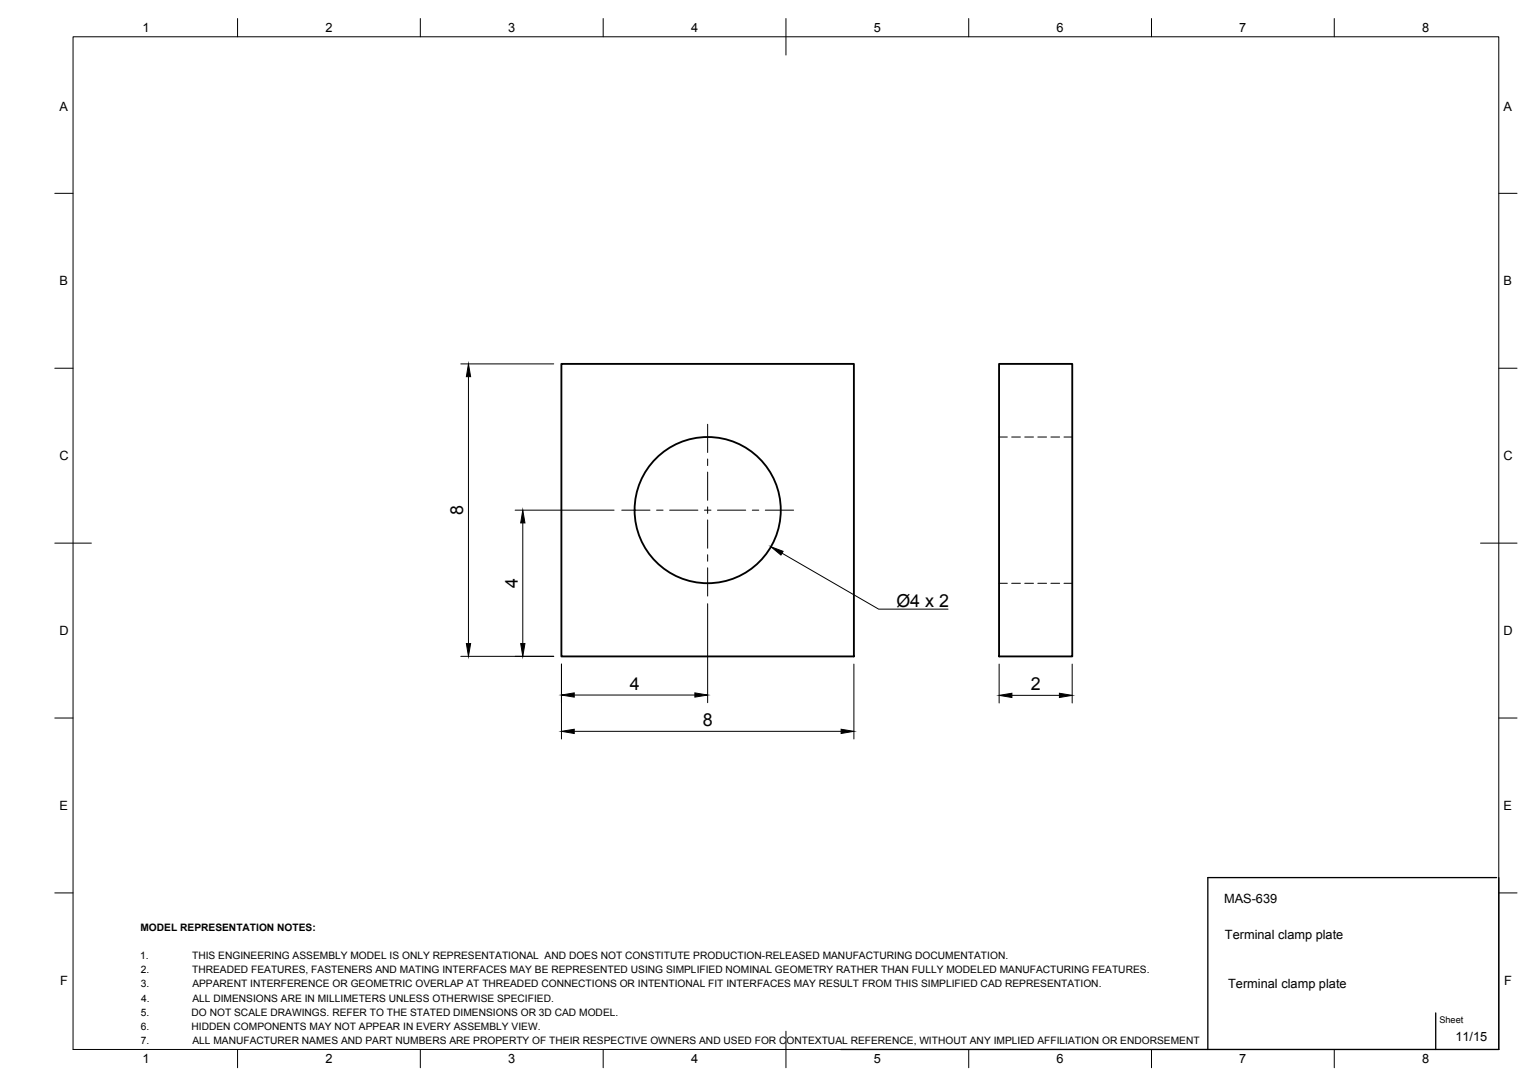
ISO-10303-21;
HEADER;
/* Generated by software containing ST-Developer
 * from STEP Tools, Inc. (www.steptools.com) 
 */

FILE_DESCRIPTION(
/* description */ ('Independent maintained push-to-latch/pull-to-reset mushroom-operator 
CAD. Two opposed spring-loaded ball detents in turned circular seats b
ias both travel stops; direct normally-closed bridge opens6mm when pre
ssed. Rounded palm/pull rim, captured head screw, removable detent clo
sures, native Coil spring families, insulated shared terminals and ord
inary machining features. Manual geometric states and ideal same-mater
ial spring-energy direction only; no electrical/safety certification, 
force/contact dynamics, wear, load or life rating. Requested blue/gray
 visual palette, not safety identification. External wiring/anchors an
d application engineering omitted.'),
/* implementation_level */ '2;1');

FILE_NAME(
/* name */ 'Terminal clamp plate.step',
/* time_stamp */ '2026-11-08T17:54:26-08:00',
/* author */ (''),
/* organization */ (''),
/* preprocessor_version */ 'ST-DEVELOPER v20.2',
/* originating_system */ 'Autodesk Translation Framework v15.17.0.0',
/* authorisation */ '');

FILE_SCHEMA (('AUTOMOTIVE_DESIGN { 1 0 10303 214 3 1 1 }'));
ENDSEC;

DATA;
#10=MECHANICAL_DESIGN_GEOMETRIC_PRESENTATION_REPRESENTATION('',(#199),#43980);
#165=SHAPE_REPRESENTATION_RELATIONSHIP('SRR','None',#44065,#182);
#182=ADVANCED_BREP_SHAPE_REPRESENTATION('',(#216),#43972);
#199=STYLED_ITEM('',(#44157),#216);
#216=MANIFOLD_SOLID_BREP('Body1',#11240);
#320=FACE_BOUND('',#1624,.T.);
#321=FACE_BOUND('',#1626,.T.);
#433=PLANE('',#12029);
#434=PLANE('',#12030);
#435=PLANE('',#12031);
#436=PLANE('',#12032);
#437=PLANE('',#12033);
#438=PLANE('',#12034);
#934=FACE_OUTER_BOUND('',#1618,.T.);
#935=FACE_OUTER_BOUND('',#1619,.T.);
#936=FACE_OUTER_BOUND('',#1620,.T.);
#937=FACE_OUTER_BOUND('',#1621,.T.);
#938=FACE_OUTER_BOUND('',#1622,.T.);
#939=FACE_OUTER_BOUND('',#1623,.T.);
#940=FACE_OUTER_BOUND('',#1625,.T.);
#1618=EDGE_LOOP('',(#9293,#9294,#9295,#9296));
#1619=EDGE_LOOP('',(#9297,#9298,#9299,#9300));
#1620=EDGE_LOOP('',(#9301,#9302,#9303,#9304));
#1621=EDGE_LOOP('',(#9305,#9306,#9307,#9308));
#1622=EDGE_LOOP('',(#9309,#9310,#9311,#9312));
#1623=EDGE_LOOP('',(#9313,#9314,#9315,#9316));
#1624=EDGE_LOOP('',(#9317));
#1625=EDGE_LOOP('',(#9318,#9319,#9320,#9321));
#1626=EDGE_LOOP('',(#9322));
#1955=CIRCLE('',#12027,0.2);
#1956=CIRCLE('',#12028,0.2);
#3275=LINE('',#35863,#3907);
#3276=LINE('',#35868,#3908);
#3277=LINE('',#35870,#3909);
#3278=LINE('',#35872,#3910);
#3279=LINE('',#35873,#3911);
#3280=LINE('',#35876,#3912);
#3281=LINE('',#35878,#3913);
#3282=LINE('',#35879,#3914);
#3283=LINE('',#35882,#3915);
#3284=LINE('',#35884,#3916);
#3285=LINE('',#35885,#3917);
#3286=LINE('',#35887,#3918);
#3287=LINE('',#35888,#3919);
#3907=VECTOR('',#13896,0.2);
#3908=VECTOR('',#13901,1.);
#3909=VECTOR('',#13902,1.);
#3910=VECTOR('',#13903,1.);
#3911=VECTOR('',#13904,1.);
#3912=VECTOR('',#13907,1.);
#3913=VECTOR('',#13908,1.);
#3914=VECTOR('',#13909,1.);
#3915=VECTOR('',#13912,1.);
#3916=VECTOR('',#13913,1.);
#3917=VECTOR('',#13914,1.);
#3918=VECTOR('',#13917,1.);
#3919=VECTOR('',#13918,1.);
#4902=VERTEX_POINT('',#35860);
#4903=VERTEX_POINT('',#35862);
#4904=VERTEX_POINT('',#35866);
#4905=VERTEX_POINT('',#35867);
#4906=VERTEX_POINT('',#35869);
#4907=VERTEX_POINT('',#35871);
#4908=VERTEX_POINT('',#35875);
#4909=VERTEX_POINT('',#35877);
#4910=VERTEX_POINT('',#35881);
#4911=VERTEX_POINT('',#35883);
#6416=EDGE_CURVE('',#4902,#4902,#1955,.T.);
#6417=EDGE_CURVE('',#4902,#4903,#3275,.T.);
#6418=EDGE_CURVE('',#4903,#4903,#1956,.T.);
#6419=EDGE_CURVE('',#4904,#4905,#3276,.T.);
#6420=EDGE_CURVE('',#4905,#4906,#3277,.T.);
#6421=EDGE_CURVE('',#4907,#4906,#3278,.T.);
#6422=EDGE_CURVE('',#4904,#4907,#3279,.T.);
#6423=EDGE_CURVE('',#4908,#4904,#3280,.T.);
#6424=EDGE_CURVE('',#4909,#4907,#3281,.T.);
#6425=EDGE_CURVE('',#4908,#4909,#3282,.T.);
#6426=EDGE_CURVE('',#4910,#4908,#3283,.T.);
#6427=EDGE_CURVE('',#4911,#4909,#3284,.T.);
#6428=EDGE_CURVE('',#4910,#4911,#3285,.T.);
#6429=EDGE_CURVE('',#4905,#4910,#3286,.T.);
#6430=EDGE_CURVE('',#4906,#4911,#3287,.T.);
#9293=ORIENTED_EDGE('',*,*,#6416,.F.);
#9294=ORIENTED_EDGE('',*,*,#6417,.T.);
#9295=ORIENTED_EDGE('',*,*,#6418,.F.);
#9296=ORIENTED_EDGE('',*,*,#6417,.F.);
#9297=ORIENTED_EDGE('',*,*,#6419,.T.);
#9298=ORIENTED_EDGE('',*,*,#6420,.T.);
#9299=ORIENTED_EDGE('',*,*,#6421,.F.);
#9300=ORIENTED_EDGE('',*,*,#6422,.F.);
#9301=ORIENTED_EDGE('',*,*,#6423,.T.);
#9302=ORIENTED_EDGE('',*,*,#6422,.T.);
#9303=ORIENTED_EDGE('',*,*,#6424,.F.);
#9304=ORIENTED_EDGE('',*,*,#6425,.F.);
#9305=ORIENTED_EDGE('',*,*,#6426,.T.);
#9306=ORIENTED_EDGE('',*,*,#6425,.T.);
#9307=ORIENTED_EDGE('',*,*,#6427,.F.);
#9308=ORIENTED_EDGE('',*,*,#6428,.F.);
#9309=ORIENTED_EDGE('',*,*,#6429,.T.);
#9310=ORIENTED_EDGE('',*,*,#6428,.T.);
#9311=ORIENTED_EDGE('',*,*,#6430,.F.);
#9312=ORIENTED_EDGE('',*,*,#6420,.F.);
#9313=ORIENTED_EDGE('',*,*,#6430,.T.);
#9314=ORIENTED_EDGE('',*,*,#6427,.T.);
#9315=ORIENTED_EDGE('',*,*,#6424,.T.);
#9316=ORIENTED_EDGE('',*,*,#6421,.T.);
#9317=ORIENTED_EDGE('',*,*,#6416,.T.);
#9318=ORIENTED_EDGE('',*,*,#6429,.F.);
#9319=ORIENTED_EDGE('',*,*,#6419,.F.);
#9320=ORIENTED_EDGE('',*,*,#6423,.F.);
#9321=ORIENTED_EDGE('',*,*,#6426,.F.);
#9322=ORIENTED_EDGE('',*,*,#6418,.T.);
#10502=CYLINDRICAL_SURFACE('',#12026,0.2);
#11059=ADVANCED_FACE('',(#934),#10502,.F.);
#11060=ADVANCED_FACE('',(#935),#433,.T.);
#11061=ADVANCED_FACE('',(#936),#434,.T.);
#11062=ADVANCED_FACE('',(#937),#435,.T.);
#11063=ADVANCED_FACE('',(#938),#436,.T.);
#11064=ADVANCED_FACE('',(#939,#320),#437,.T.);
#11065=ADVANCED_FACE('',(#940,#321),#438,.F.);
#11240=CLOSED_SHELL('',(#11059,#11060,#11061,#11062,#11063,#11064,#11065));
#12025=AXIS2_PLACEMENT_3D('',#35858,#13890,#13891);
#12026=AXIS2_PLACEMENT_3D('',#35859,#13892,#13893);
#12027=AXIS2_PLACEMENT_3D('',#35861,#13894,#13895);
#12028=AXIS2_PLACEMENT_3D('',#35864,#13897,#13898);
#12029=AXIS2_PLACEMENT_3D('',#35865,#13899,#13900);
#12030=AXIS2_PLACEMENT_3D('',#35874,#13905,#13906);
#12031=AXIS2_PLACEMENT_3D('',#35880,#13910,#13911);
#12032=AXIS2_PLACEMENT_3D('',#35886,#13915,#13916);
#12033=AXIS2_PLACEMENT_3D('',#35889,#13919,#13920);
#12034=AXIS2_PLACEMENT_3D('',#35890,#13921,#13922);
#13890=DIRECTION('axis',(0.,0.,1.));
#13891=DIRECTION('refdir',(1.,0.,0.));
#13892=DIRECTION('center_axis',(0.,0.,-1.));
#13893=DIRECTION('ref_axis',(1.,0.,0.));
#13894=DIRECTION('center_axis',(0.,0.,-1.));
#13895=DIRECTION('ref_axis',(1.,0.,0.));
#13896=DIRECTION('',(0.,0.,-1.));
#13897=DIRECTION('center_axis',(0.,0.,1.));
#13898=DIRECTION('ref_axis',(1.,0.,0.));
#13899=DIRECTION('center_axis',(0.,1.,0.));
#13900=DIRECTION('ref_axis',(-1.,0.,0.));
#13901=DIRECTION('',(-1.,0.,0.));
#13902=DIRECTION('',(0.,0.,1.));
#13903=DIRECTION('',(-1.,0.,0.));
#13904=DIRECTION('',(0.,0.,1.));
#13905=DIRECTION('center_axis',(1.,0.,0.));
#13906=DIRECTION('ref_axis',(0.,1.,0.));
#13907=DIRECTION('',(0.,1.,0.));
#13908=DIRECTION('',(0.,1.,0.));
#13909=DIRECTION('',(0.,0.,1.));
#13910=DIRECTION('center_axis',(0.,-1.,0.));
#13911=DIRECTION('ref_axis',(1.,0.,0.));
#13912=DIRECTION('',(1.,0.,0.));
#13913=DIRECTION('',(1.,0.,0.));
#13914=DIRECTION('',(0.,0.,1.));
#13915=DIRECTION('center_axis',(-1.,0.,0.));
#13916=DIRECTION('ref_axis',(0.,-1.,0.));
#13917=DIRECTION('',(0.,-1.,0.));
#13918=DIRECTION('',(0.,-1.,0.));
#13919=DIRECTION('center_axis',(0.,0.,1.));
#13920=DIRECTION('ref_axis',(1.,0.,0.));
#13921=DIRECTION('center_axis',(0.,0.,1.));
#13922=DIRECTION('ref_axis',(1.,0.,0.));
#35858=CARTESIAN_POINT('',(0.,0.,0.));
#35859=CARTESIAN_POINT('Origin',(0.,0.,4.1));
#35860=CARTESIAN_POINT('',(-0.2,2.44929359829471E-17,4.2));
#35861=CARTESIAN_POINT('Origin',(0.,0.,4.2));
#35862=CARTESIAN_POINT('',(-0.2,2.44929359829471E-17,4.));
#35863=CARTESIAN_POINT('',(-0.2,2.44929359829471E-17,4.1));
#35864=CARTESIAN_POINT('Origin',(0.,0.,4.));
#35865=CARTESIAN_POINT('Origin',(0.4,0.4,4.));
#35866=CARTESIAN_POINT('',(0.4,0.4,4.));
#35867=CARTESIAN_POINT('',(-0.4,0.4,4.));
#35868=CARTESIAN_POINT('',(0.4,0.4,4.));
#35869=CARTESIAN_POINT('',(-0.4,0.4,4.2));
#35870=CARTESIAN_POINT('',(-0.4,0.4,4.));
#35871=CARTESIAN_POINT('',(0.4,0.4,4.2));
#35872=CARTESIAN_POINT('',(0.4,0.4,4.2));
#35873=CARTESIAN_POINT('',(0.4,0.4,4.));
#35874=CARTESIAN_POINT('Origin',(0.4,-0.4,4.));
#35875=CARTESIAN_POINT('',(0.4,-0.4,4.));
#35876=CARTESIAN_POINT('',(0.4,-0.4,4.));
#35877=CARTESIAN_POINT('',(0.4,-0.4,4.2));
#35878=CARTESIAN_POINT('',(0.4,-0.4,4.2));
#35879=CARTESIAN_POINT('',(0.4,-0.4,4.));
#35880=CARTESIAN_POINT('Origin',(-0.4,-0.4,4.));
#35881=CARTESIAN_POINT('',(-0.4,-0.4,4.));
#35882=CARTESIAN_POINT('',(-0.4,-0.4,4.));
#35883=CARTESIAN_POINT('',(-0.4,-0.4,4.2));
#35884=CARTESIAN_POINT('',(-0.4,-0.4,4.2));
#35885=CARTESIAN_POINT('',(-0.4,-0.4,4.));
#35886=CARTESIAN_POINT('Origin',(-0.4,0.4,4.));
#35887=CARTESIAN_POINT('',(-0.4,0.4,4.));
#35888=CARTESIAN_POINT('',(-0.4,0.4,4.2));
#35889=CARTESIAN_POINT('Origin',(0.,0.,4.2));
#35890=CARTESIAN_POINT('Origin',(0.,0.,4.));
#43953=UNCERTAINTY_MEASURE_WITH_UNIT(LENGTH_MEASURE(0.001),#43981,
'DISTANCE_ACCURACY_VALUE',
'Maximum model space distance between geometric entities at asserted c
onnectivities');
#43961=UNCERTAINTY_MEASURE_WITH_UNIT(LENGTH_MEASURE(0.001),#43981,
'DISTANCE_ACCURACY_VALUE',
'Maximum model space distance between geometric entities at asserted c
onnectivities');
#43972=(
GEOMETRIC_REPRESENTATION_CONTEXT(3)
GLOBAL_UNCERTAINTY_ASSIGNED_CONTEXT((#43953))
GLOBAL_UNIT_ASSIGNED_CONTEXT((#43981,#43983,#43984))
REPRESENTATION_CONTEXT('','3D')
);
#43980=(
GEOMETRIC_REPRESENTATION_CONTEXT(3)
GLOBAL_UNCERTAINTY_ASSIGNED_CONTEXT((#43961))
GLOBAL_UNIT_ASSIGNED_CONTEXT((#43981,#43983,#43984))
REPRESENTATION_CONTEXT('','3D')
);
#43981=(
LENGTH_UNIT()
NAMED_UNIT(*)
SI_UNIT(.CENTI.,.METRE.)
);
#43983=(
NAMED_UNIT(*)
PLANE_ANGLE_UNIT()
SI_UNIT($,.RADIAN.)
);
#43984=(
NAMED_UNIT(*)
SI_UNIT($,.STERADIAN.)
SOLID_ANGLE_UNIT()
);
#43995=SHAPE_DEFINITION_REPRESENTATION(#44013,#44065);
#44013=PRODUCT_DEFINITION_SHAPE('',$,#44084);
#44065=SHAPE_REPRESENTATION('',(#12025),#43972);
#44073=PRODUCT_DEFINITION_CONTEXT('part definition',#44129,'design');
#44084=PRODUCT_DEFINITION('Terminal clamp plate','Terminal clamp plate',
#44102,#44073);
#44102=PRODUCT_DEFINITION_FORMATION('',$,#44141);
#44129=APPLICATION_CONTEXT(
'Core Data for Automotive Mechanical Design Process');
#44130=PRODUCT_CONTEXT('part definition',#44129,'mechanical');
#44141=PRODUCT('Terminal clamp plate','Terminal clamp plate',$,(#44130));
#44157=PRESENTATION_STYLE_ASSIGNMENT((#44169));
#44169=SURFACE_STYLE_USAGE(.BOTH.,#44181);
#44181=SURFACE_SIDE_STYLE('',(#44193));
#44193=SURFACE_STYLE_FILL_AREA(#44205);
#44205=FILL_AREA_STYLE('Clamp gray',(#44217));
#44217=FILL_AREA_STYLE_COLOUR('Clamp gray',#44229);
#44229=COLOUR_RGB('Clamp gray',0.407843137254902,0.447058823529412,0.498039215686275);
ENDSEC;
END-ISO-10303-21;
